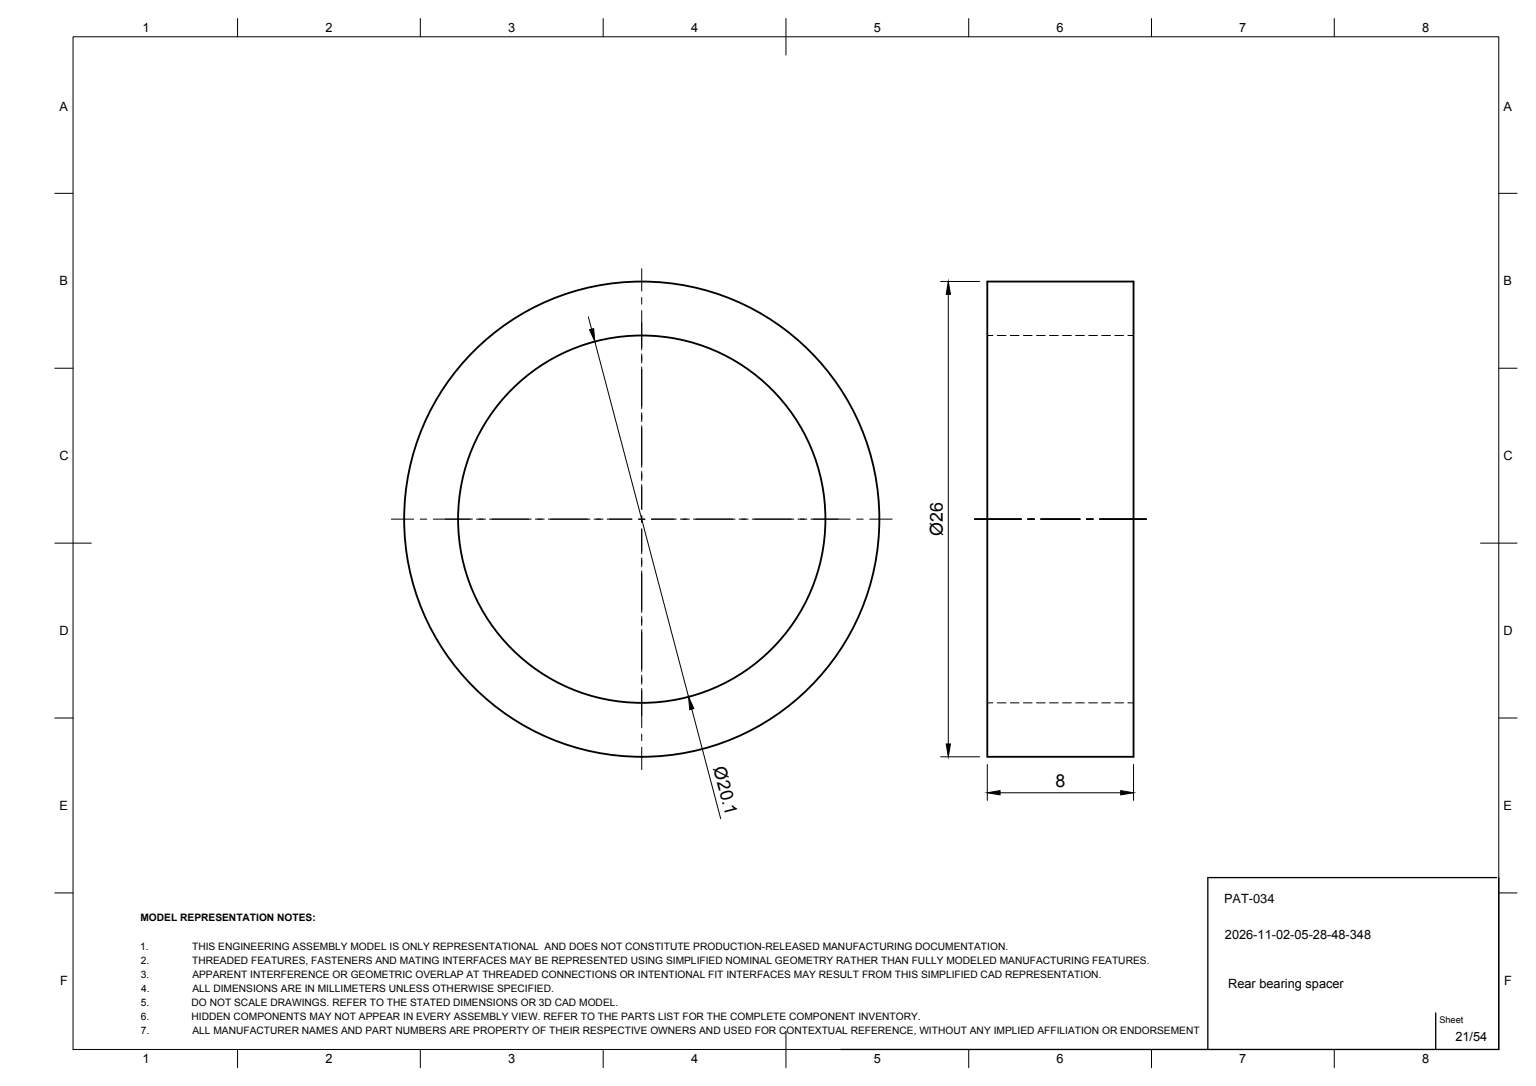
ISO-10303-21;
HEADER;
/* Generated by software containing ST-Developer
 * from STEP Tools, Inc. (www.steptools.com) 
 */

FILE_DESCRIPTION(
/* description */ ('Fatigue rig crank-slider'),
/* implementation_level */ '2;1');

FILE_NAME(
/* name */ 'Rear bearing spacer.step',
/* time_stamp */ '2026-10-28T03:24:50-07:00',
/* author */ (''),
/* organization */ (''),
/* preprocessor_version */ 'ST-DEVELOPER v20.2',
/* originating_system */ 'Autodesk Translation Framework v15.17.0.0',
/* authorisation */ '');

FILE_SCHEMA (('AUTOMOTIVE_DESIGN { 1 0 10303 214 3 1 1 }'));
ENDSEC;

DATA;
#10=MECHANICAL_DESIGN_GEOMETRIC_PRESENTATION_REPRESENTATION('',(#607),#16911);
#506=SHAPE_REPRESENTATION_RELATIONSHIP('SRR','None',#17147,#556);
#556=ADVANCED_BREP_SHAPE_REPRESENTATION('',(#664),#16876);
#607=STYLED_ITEM('',(#17487),#664);
#664=MANIFOLD_SOLID_BREP('Body1',#8900);
#829=FACE_BOUND('',#2113,.T.);
#830=FACE_BOUND('',#2115,.T.);
#1041=PLANE('',#9949);
#1042=PLANE('',#9950);
#1458=FACE_OUTER_BOUND('',#2110,.T.);
#1459=FACE_OUTER_BOUND('',#2111,.T.);
#1460=FACE_OUTER_BOUND('',#2112,.T.);
#1461=FACE_OUTER_BOUND('',#2114,.T.);
#2110=EDGE_LOOP('',(#7014,#7015,#7016,#7017));
#2111=EDGE_LOOP('',(#7018,#7019,#7020,#7021));
#2112=EDGE_LOOP('',(#7022));
#2113=EDGE_LOOP('',(#7023));
#2114=EDGE_LOOP('',(#7024));
#2115=EDGE_LOOP('',(#7025));
#2754=LINE('',#15011,#3400);
#2755=LINE('',#15017,#3401);
#3400=VECTOR('',#11764,1.005);
#3401=VECTOR('',#11771,1.3);
#3935=CIRCLE('',#9944,1.005);
#3936=CIRCLE('',#9945,1.005);
#3937=CIRCLE('',#9947,1.3);
#3938=CIRCLE('',#9948,1.3);
#4497=VERTEX_POINT('',#15008);
#4498=VERTEX_POINT('',#15010);
#4499=VERTEX_POINT('',#15014);
#4500=VERTEX_POINT('',#15016);
#5405=EDGE_CURVE('',#4497,#4497,#3935,.T.);
#5406=EDGE_CURVE('',#4497,#4498,#2754,.T.);
#5407=EDGE_CURVE('',#4498,#4498,#3936,.T.);
#5408=EDGE_CURVE('',#4499,#4499,#3937,.T.);
#5409=EDGE_CURVE('',#4499,#4500,#2755,.T.);
#5410=EDGE_CURVE('',#4500,#4500,#3938,.T.);
#7014=ORIENTED_EDGE('',*,*,#5405,.F.);
#7015=ORIENTED_EDGE('',*,*,#5406,.T.);
#7016=ORIENTED_EDGE('',*,*,#5407,.T.);
#7017=ORIENTED_EDGE('',*,*,#5406,.F.);
#7018=ORIENTED_EDGE('',*,*,#5408,.F.);
#7019=ORIENTED_EDGE('',*,*,#5409,.T.);
#7020=ORIENTED_EDGE('',*,*,#5410,.T.);
#7021=ORIENTED_EDGE('',*,*,#5409,.F.);
#7022=ORIENTED_EDGE('',*,*,#5408,.T.);
#7023=ORIENTED_EDGE('',*,*,#5405,.T.);
#7024=ORIENTED_EDGE('',*,*,#5410,.F.);
#7025=ORIENTED_EDGE('',*,*,#5407,.F.);
#8284=CYLINDRICAL_SURFACE('',#9943,1.005);
#8285=CYLINDRICAL_SURFACE('',#9946,1.3);
#8596=ADVANCED_FACE('',(#1458),#8284,.F.);
#8597=ADVANCED_FACE('',(#1459),#8285,.T.);
#8598=ADVANCED_FACE('',(#1460,#829),#1041,.T.);
#8599=ADVANCED_FACE('',(#1461,#830),#1042,.F.);
#8900=CLOSED_SHELL('',(#8596,#8597,#8598,#8599));
#9942=AXIS2_PLACEMENT_3D('',#15006,#11758,#11759);
#9943=AXIS2_PLACEMENT_3D('',#15007,#11760,#11761);
#9944=AXIS2_PLACEMENT_3D('',#15009,#11762,#11763);
#9945=AXIS2_PLACEMENT_3D('',#15012,#11765,#11766);
#9946=AXIS2_PLACEMENT_3D('',#15013,#11767,#11768);
#9947=AXIS2_PLACEMENT_3D('',#15015,#11769,#11770);
#9948=AXIS2_PLACEMENT_3D('',#15018,#11772,#11773);
#9949=AXIS2_PLACEMENT_3D('',#15019,#11774,#11775);
#9950=AXIS2_PLACEMENT_3D('',#15020,#11776,#11777);
#11758=DIRECTION('axis',(0.,0.,1.));
#11759=DIRECTION('refdir',(1.,0.,0.));
#11760=DIRECTION('center_axis',(0.,1.,0.));
#11761=DIRECTION('ref_axis',(1.,0.,0.));
#11762=DIRECTION('center_axis',(0.,-1.,0.));
#11763=DIRECTION('ref_axis',(1.,0.,0.));
#11764=DIRECTION('',(0.,-1.,0.));
#11765=DIRECTION('center_axis',(0.,-1.,0.));
#11766=DIRECTION('ref_axis',(1.,0.,0.));
#11767=DIRECTION('center_axis',(0.,1.,0.));
#11768=DIRECTION('ref_axis',(1.,0.,0.));
#11769=DIRECTION('center_axis',(0.,1.,0.));
#11770=DIRECTION('ref_axis',(1.,0.,0.));
#11771=DIRECTION('',(0.,-1.,0.));
#11772=DIRECTION('center_axis',(0.,1.,0.));
#11773=DIRECTION('ref_axis',(1.,0.,0.));
#11774=DIRECTION('center_axis',(0.,1.,0.));
#11775=DIRECTION('ref_axis',(1.,0.,0.));
#11776=DIRECTION('center_axis',(0.,1.,0.));
#11777=DIRECTION('ref_axis',(1.,0.,0.));
#15006=CARTESIAN_POINT('',(0.,0.,0.));
#15007=CARTESIAN_POINT('Origin',(0.,-16.65,12.));
#15008=CARTESIAN_POINT('',(-1.005,-15.85,12.));
#15009=CARTESIAN_POINT('Origin',(0.,-15.85,12.));
#15010=CARTESIAN_POINT('',(-1.005,-16.65,12.));
#15011=CARTESIAN_POINT('',(-1.005,-16.65,12.));
#15012=CARTESIAN_POINT('Origin',(0.,-16.65,12.));
#15013=CARTESIAN_POINT('Origin',(0.,-16.65,12.));
#15014=CARTESIAN_POINT('',(-1.3,-15.85,12.));
#15015=CARTESIAN_POINT('Origin',(0.,-15.85,12.));
#15016=CARTESIAN_POINT('',(-1.3,-16.65,12.));
#15017=CARTESIAN_POINT('',(-1.3,-16.65,12.));
#15018=CARTESIAN_POINT('Origin',(0.,-16.65,12.));
#15019=CARTESIAN_POINT('Origin',(0.,-15.85,12.));
#15020=CARTESIAN_POINT('Origin',(0.,-16.65,12.));
#16817=UNCERTAINTY_MEASURE_WITH_UNIT(LENGTH_MEASURE(0.001),#16912,
'DISTANCE_ACCURACY_VALUE',
'Maximum model space distance between geometric entities at asserted c
onnectivities');
#16852=UNCERTAINTY_MEASURE_WITH_UNIT(LENGTH_MEASURE(0.001),#16912,
'DISTANCE_ACCURACY_VALUE',
'Maximum model space distance between geometric entities at asserted c
onnectivities');
#16876=(
GEOMETRIC_REPRESENTATION_CONTEXT(3)
GLOBAL_UNCERTAINTY_ASSIGNED_CONTEXT((#16817))
GLOBAL_UNIT_ASSIGNED_CONTEXT((#16912,#16914,#16915))
REPRESENTATION_CONTEXT('','3D')
);
#16911=(
GEOMETRIC_REPRESENTATION_CONTEXT(3)
GLOBAL_UNCERTAINTY_ASSIGNED_CONTEXT((#16852))
GLOBAL_UNIT_ASSIGNED_CONTEXT((#16912,#16914,#16915))
REPRESENTATION_CONTEXT('','3D')
);
#16912=(
LENGTH_UNIT()
NAMED_UNIT(*)
SI_UNIT(.CENTI.,.METRE.)
);
#16914=(
NAMED_UNIT(*)
PLANE_ANGLE_UNIT()
SI_UNIT($,.RADIAN.)
);
#16915=(
NAMED_UNIT(*)
SI_UNIT($,.STERADIAN.)
SOLID_ANGLE_UNIT()
);
#16939=SHAPE_DEFINITION_REPRESENTATION(#16999,#17147);
#16999=PRODUCT_DEFINITION_SHAPE('',$,#17206);
#17147=SHAPE_REPRESENTATION('',(#9942),#16876);
#17182=PRODUCT_DEFINITION_CONTEXT('part definition',#17358,'design');
#17206=PRODUCT_DEFINITION('Rear bearing spacer','Rear bearing spacer',#17264,
#17182);
#17264=PRODUCT_DEFINITION_FORMATION('',$,#17383);
#17358=APPLICATION_CONTEXT(
'Core Data for Automotive Mechanical Design Process');
#17359=PRODUCT_CONTEXT('part definition',#17358,'mechanical');
#17383=PRODUCT('Rear bearing spacer','Rear bearing spacer',
'Rear bearing spacer',(#17359));
#17481=COLOUR_RGB('Grey',0.48,0.52,0.57);
#17482=FILL_AREA_STYLE_COLOUR('',#17481);
#17483=FILL_AREA_STYLE('',(#17482));
#17484=SURFACE_STYLE_FILL_AREA(#17483);
#17485=SURFACE_SIDE_STYLE('',(#17484));
#17486=SURFACE_STYLE_USAGE(.BOTH.,#17485);
#17487=PRESENTATION_STYLE_ASSIGNMENT((#17486));
ENDSEC;
END-ISO-10303-21;
